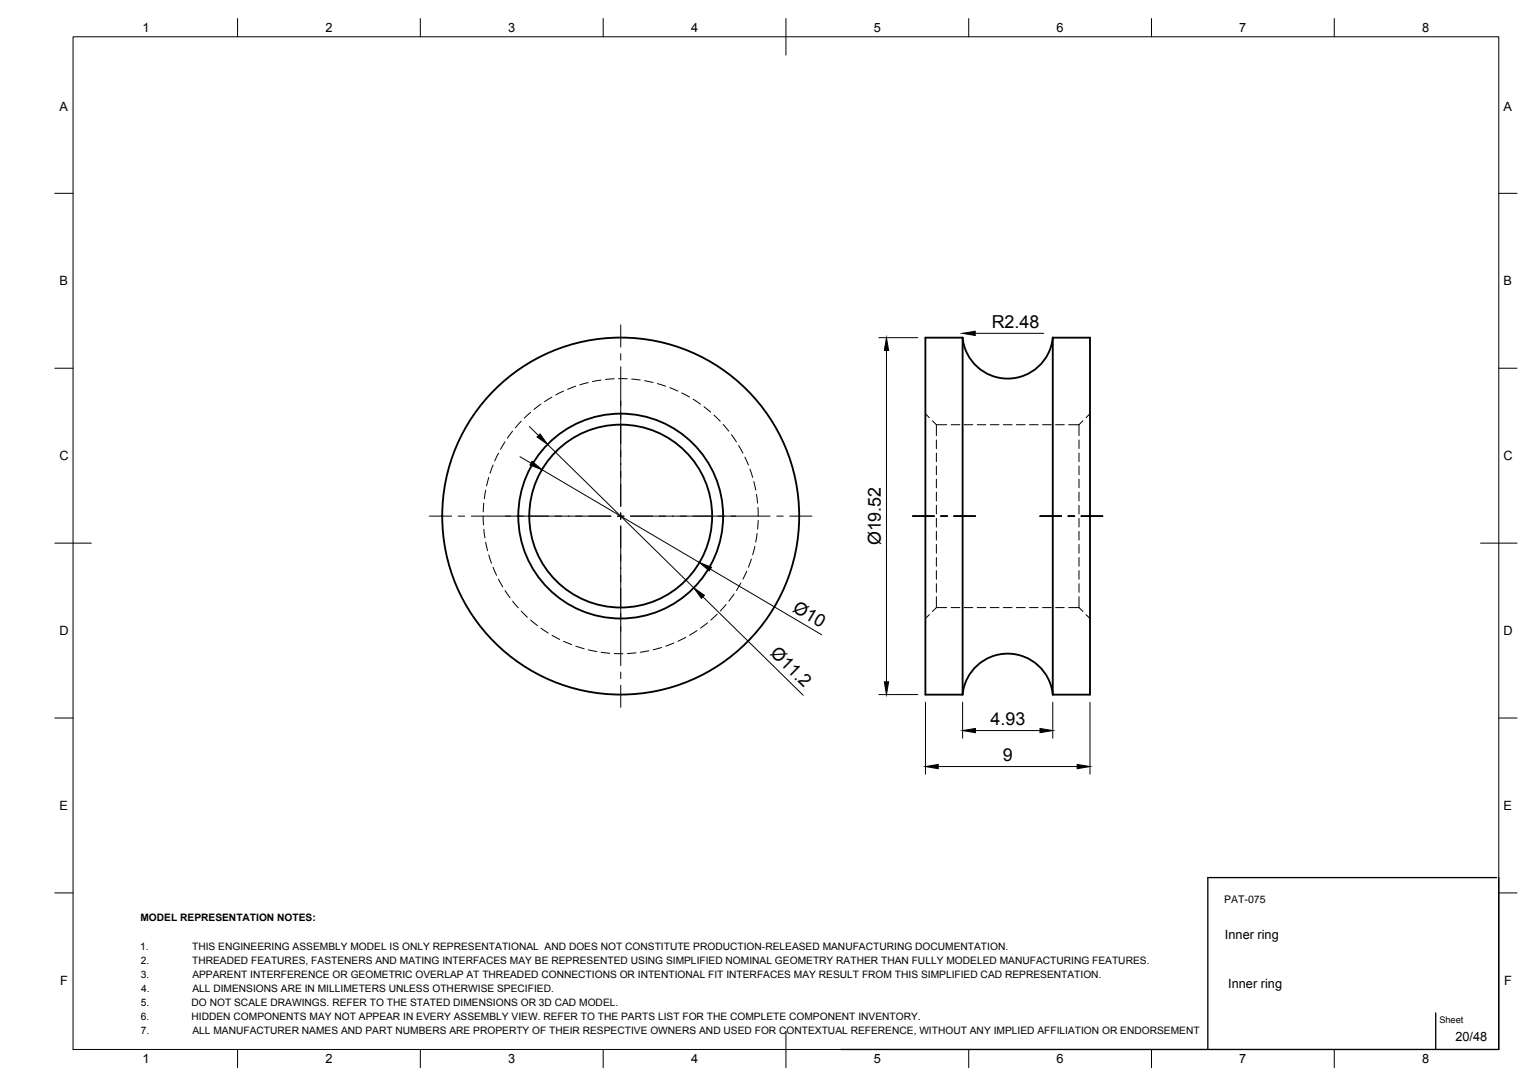
ISO-10303-21;
HEADER;
/* Generated by software containing ST-Developer
 * from STEP Tools, Inc. (www.steptools.com) 
 */

FILE_DESCRIPTION(
/* description */ ('Over-Centre Plunger Toggle Clamp on Slotted Fixture Frame'),
/* implementation_level */ '2;1');

FILE_NAME(
/* name */ 
'Inner ring.step',
/* time_stamp */ '2026-10-28T03:23:24-07:00',
/* author */ (''),
/* organization */ (''),
/* preprocessor_version */ 'ST-DEVELOPER v20.2',
/* originating_system */ 'Autodesk Translation Framework v15.17.0.0',
/* authorisation */ '');

FILE_SCHEMA (('AUTOMOTIVE_DESIGN { 1 0 10303 214 3 1 1 }'));
ENDSEC;

DATA;
#10=MECHANICAL_DESIGN_GEOMETRIC_PRESENTATION_REPRESENTATION('',(#529),#15212);
#395=TOROIDAL_SURFACE('',#9166,1.,0.247676);
#409=CONICAL_SURFACE('',#9177,0.53,0.785398163397448);
#410=CONICAL_SURFACE('',#9184,0.53,0.785398163397448);
#445=SHAPE_REPRESENTATION_RELATIONSHIP('SRR','None',#15420,#487);
#487=ADVANCED_BREP_SHAPE_REPRESENTATION('',(#579),#15182);
#529=STYLED_ITEM('',(#15719),#579);
#579=MANIFOLD_SOLID_BREP('Body1',#8262);
#720=FACE_BOUND('',#1918,.T.);
#721=FACE_BOUND('',#1921,.T.);
#938=PLANE('',#9179);
#939=PLANE('',#9182);
#1318=FACE_OUTER_BOUND('',#1913,.T.);
#1319=FACE_OUTER_BOUND('',#1914,.T.);
#1320=FACE_OUTER_BOUND('',#1915,.T.);
#1321=FACE_OUTER_BOUND('',#1916,.T.);
#1322=FACE_OUTER_BOUND('',#1917,.T.);
#1323=FACE_OUTER_BOUND('',#1919,.T.);
#1324=FACE_OUTER_BOUND('',#1920,.T.);
#1325=FACE_OUTER_BOUND('',#1922,.T.);
#1913=EDGE_LOOP('',(#6629,#6630,#6631,#6632,#6633,#6634));
#1914=EDGE_LOOP('',(#6635,#6636,#6637,#6638,#6639));
#1915=EDGE_LOOP('',(#6640,#6641,#6642,#6643));
#1916=EDGE_LOOP('',(#6644,#6645,#6646,#6647));
#1917=EDGE_LOOP('',(#6648));
#1918=EDGE_LOOP('',(#6649));
#1919=EDGE_LOOP('',(#6650,#6651,#6652,#6653,#6654));
#1920=EDGE_LOOP('',(#6655));
#1921=EDGE_LOOP('',(#6656));
#1922=EDGE_LOOP('',(#6657,#6658,#6659,#6660));
#2609=LINE('',#13511,#3239);
#2610=LINE('',#13517,#3240);
#2611=LINE('',#13521,#3241);
#2612=LINE('',#13527,#3242);
#2613=LINE('',#13532,#3243);
#3239=VECTOR('',#10952,0.976185);
#3240=VECTOR('',#10959,0.5);
#3241=VECTOR('',#10964,0.53);
#3242=VECTOR('',#10973,0.976185);
#3243=VECTOR('',#10980,0.53);
#3641=CIRCLE('',#9167,0.976185);
#3642=CIRCLE('',#9168,0.976185);
#3643=CIRCLE('',#9169,0.247676);
#3644=CIRCLE('',#9170,0.976185);
#3645=CIRCLE('',#9171,0.976185);
#3646=CIRCLE('',#9173,0.976185);
#3647=CIRCLE('',#9175,0.5);
#3648=CIRCLE('',#9176,0.5);
#3649=CIRCLE('',#9178,0.56);
#3650=CIRCLE('',#9181,0.976185);
#3651=CIRCLE('',#9183,0.56);
#4211=VERTEX_POINT('',#13500);
#4212=VERTEX_POINT('',#13501);
#4213=VERTEX_POINT('',#13504);
#4214=VERTEX_POINT('',#13506);
#4215=VERTEX_POINT('',#13510);
#4216=VERTEX_POINT('',#13514);
#4217=VERTEX_POINT('',#13516);
#4218=VERTEX_POINT('',#13520);
#4219=VERTEX_POINT('',#13525);
#4220=VERTEX_POINT('',#13529);
#5075=EDGE_CURVE('',#4211,#4212,#3641,.T.);
#5076=EDGE_CURVE('',#4212,#4211,#3642,.T.);
#5077=EDGE_CURVE('',#4212,#4213,#3643,.T.);
#5078=EDGE_CURVE('',#4214,#4213,#3644,.T.);
#5079=EDGE_CURVE('',#4213,#4214,#3645,.T.);
#5080=EDGE_CURVE('',#4214,#4215,#2609,.T.);
#5081=EDGE_CURVE('',#4215,#4215,#3646,.T.);
#5082=EDGE_CURVE('',#4216,#4216,#3647,.T.);
#5083=EDGE_CURVE('',#4216,#4217,#2610,.T.);
#5084=EDGE_CURVE('',#4217,#4217,#3648,.T.);
#5085=EDGE_CURVE('',#4217,#4218,#2611,.T.);
#5086=EDGE_CURVE('',#4218,#4218,#3649,.T.);
#5087=EDGE_CURVE('',#4219,#4219,#3650,.T.);
#5088=EDGE_CURVE('',#4219,#4211,#2612,.T.);
#5089=EDGE_CURVE('',#4220,#4220,#3651,.T.);
#5090=EDGE_CURVE('',#4220,#4216,#2613,.T.);
#6629=ORIENTED_EDGE('',*,*,#5075,.F.);
#6630=ORIENTED_EDGE('',*,*,#5076,.F.);
#6631=ORIENTED_EDGE('',*,*,#5077,.T.);
#6632=ORIENTED_EDGE('',*,*,#5078,.F.);
#6633=ORIENTED_EDGE('',*,*,#5079,.F.);
#6634=ORIENTED_EDGE('',*,*,#5077,.F.);
#6635=ORIENTED_EDGE('',*,*,#5078,.T.);
#6636=ORIENTED_EDGE('',*,*,#5079,.T.);
#6637=ORIENTED_EDGE('',*,*,#5080,.T.);
#6638=ORIENTED_EDGE('',*,*,#5081,.T.);
#6639=ORIENTED_EDGE('',*,*,#5080,.F.);
#6640=ORIENTED_EDGE('',*,*,#5082,.T.);
#6641=ORIENTED_EDGE('',*,*,#5083,.T.);
#6642=ORIENTED_EDGE('',*,*,#5084,.F.);
#6643=ORIENTED_EDGE('',*,*,#5083,.F.);
#6644=ORIENTED_EDGE('',*,*,#5084,.T.);
#6645=ORIENTED_EDGE('',*,*,#5085,.T.);
#6646=ORIENTED_EDGE('',*,*,#5086,.F.);
#6647=ORIENTED_EDGE('',*,*,#5085,.F.);
#6648=ORIENTED_EDGE('',*,*,#5081,.F.);
#6649=ORIENTED_EDGE('',*,*,#5086,.T.);
#6650=ORIENTED_EDGE('',*,*,#5087,.F.);
#6651=ORIENTED_EDGE('',*,*,#5088,.T.);
#6652=ORIENTED_EDGE('',*,*,#5075,.T.);
#6653=ORIENTED_EDGE('',*,*,#5076,.T.);
#6654=ORIENTED_EDGE('',*,*,#5088,.F.);
#6655=ORIENTED_EDGE('',*,*,#5087,.T.);
#6656=ORIENTED_EDGE('',*,*,#5089,.F.);
#6657=ORIENTED_EDGE('',*,*,#5089,.T.);
#6658=ORIENTED_EDGE('',*,*,#5090,.T.);
#6659=ORIENTED_EDGE('',*,*,#5082,.F.);
#6660=ORIENTED_EDGE('',*,*,#5090,.F.);
#7689=CYLINDRICAL_SURFACE('',#9172,0.976185);
#7690=CYLINDRICAL_SURFACE('',#9174,0.5);
#7691=CYLINDRICAL_SURFACE('',#9180,0.976185);
#7990=ADVANCED_FACE('',(#1318),#395,.F.);
#7991=ADVANCED_FACE('',(#1319),#7689,.T.);
#7992=ADVANCED_FACE('',(#1320),#7690,.F.);
#7993=ADVANCED_FACE('',(#1321),#409,.F.);
#7994=ADVANCED_FACE('',(#1322,#720),#938,.T.);
#7995=ADVANCED_FACE('',(#1323),#7691,.T.);
#7996=ADVANCED_FACE('',(#1324,#721),#939,.T.);
#7997=ADVANCED_FACE('',(#1325),#410,.F.);
#8262=CLOSED_SHELL('',(#7990,#7991,#7992,#7993,#7994,#7995,#7996,#7997));
#9165=AXIS2_PLACEMENT_3D('',#13498,#10936,#10937);
#9166=AXIS2_PLACEMENT_3D('',#13499,#10938,#10939);
#9167=AXIS2_PLACEMENT_3D('',#13502,#10940,#10941);
#9168=AXIS2_PLACEMENT_3D('',#13503,#10942,#10943);
#9169=AXIS2_PLACEMENT_3D('',#13505,#10944,#10945);
#9170=AXIS2_PLACEMENT_3D('',#13507,#10946,#10947);
#9171=AXIS2_PLACEMENT_3D('',#13508,#10948,#10949);
#9172=AXIS2_PLACEMENT_3D('',#13509,#10950,#10951);
#9173=AXIS2_PLACEMENT_3D('',#13512,#10953,#10954);
#9174=AXIS2_PLACEMENT_3D('',#13513,#10955,#10956);
#9175=AXIS2_PLACEMENT_3D('',#13515,#10957,#10958);
#9176=AXIS2_PLACEMENT_3D('',#13518,#10960,#10961);
#9177=AXIS2_PLACEMENT_3D('',#13519,#10962,#10963);
#9178=AXIS2_PLACEMENT_3D('',#13522,#10965,#10966);
#9179=AXIS2_PLACEMENT_3D('',#13523,#10967,#10968);
#9180=AXIS2_PLACEMENT_3D('',#13524,#10969,#10970);
#9181=AXIS2_PLACEMENT_3D('',#13526,#10971,#10972);
#9182=AXIS2_PLACEMENT_3D('',#13528,#10974,#10975);
#9183=AXIS2_PLACEMENT_3D('',#13530,#10976,#10977);
#9184=AXIS2_PLACEMENT_3D('',#13531,#10978,#10979);
#10936=DIRECTION('axis',(0.,0.,1.));
#10937=DIRECTION('refdir',(1.,0.,0.));
#10938=DIRECTION('center_axis',(0.,-1.,0.));
#10939=DIRECTION('ref_axis',(0.,0.,-1.));
#10940=DIRECTION('center_axis',(0.,-1.,0.));
#10941=DIRECTION('ref_axis',(1.,0.,0.));
#10942=DIRECTION('center_axis',(0.,-1.,0.));
#10943=DIRECTION('ref_axis',(1.,0.,0.));
#10944=DIRECTION('center_axis',(1.,0.,1.22464679914735E-16));
#10945=DIRECTION('ref_axis',(-1.22464679914735E-16,0.,1.));
#10946=DIRECTION('center_axis',(0.,1.,0.));
#10947=DIRECTION('ref_axis',(1.,0.,0.));
#10948=DIRECTION('center_axis',(0.,1.,0.));
#10949=DIRECTION('ref_axis',(1.,0.,0.));
#10950=DIRECTION('center_axis',(0.,-1.,0.));
#10951=DIRECTION('ref_axis',(1.,0.,0.));
#10952=DIRECTION('',(0.,1.,0.));
#10953=DIRECTION('center_axis',(0.,-1.,0.));
#10954=DIRECTION('ref_axis',(1.,0.,0.));
#10955=DIRECTION('center_axis',(0.,-1.,0.));
#10956=DIRECTION('ref_axis',(1.,0.,0.));
#10957=DIRECTION('center_axis',(0.,-1.,0.));
#10958=DIRECTION('ref_axis',(1.,0.,0.));
#10959=DIRECTION('',(0.,1.,0.));
#10960=DIRECTION('center_axis',(0.,-1.,0.));
#10961=DIRECTION('ref_axis',(1.,0.,0.));
#10962=DIRECTION('center_axis',(0.,1.,0.));
#10963=DIRECTION('ref_axis',(1.,0.,0.));
#10964=DIRECTION('',(-0.707106781186547,0.707106781186548,-8.65956056235493E-17));
#10965=DIRECTION('center_axis',(0.,-1.,0.));
#10966=DIRECTION('ref_axis',(1.,0.,0.));
#10967=DIRECTION('center_axis',(0.,1.,0.));
#10968=DIRECTION('ref_axis',(0.,0.,1.));
#10969=DIRECTION('center_axis',(0.,-1.,0.));
#10970=DIRECTION('ref_axis',(1.,0.,0.));
#10971=DIRECTION('center_axis',(0.,-1.,0.));
#10972=DIRECTION('ref_axis',(1.,0.,0.));
#10973=DIRECTION('',(0.,1.,0.));
#10974=DIRECTION('center_axis',(0.,-1.,0.));
#10975=DIRECTION('ref_axis',(0.,0.,-1.));
#10976=DIRECTION('center_axis',(0.,-1.,0.));
#10977=DIRECTION('ref_axis',(1.,0.,0.));
#10978=DIRECTION('center_axis',(0.,-1.,0.));
#10979=DIRECTION('ref_axis',(1.,0.,0.));
#10980=DIRECTION('',(0.707106781186547,0.707106781186548,8.65956056235493E-17));
#13498=CARTESIAN_POINT('',(0.,0.,0.));
#13499=CARTESIAN_POINT('Origin',(0.,0.,0.));
#13500=CARTESIAN_POINT('',(-0.976185,-0.246528389340863,-1.19548183562566E-16));
#13501=CARTESIAN_POINT('',(-1.19548183562566E-16,-0.246528389340863,0.976185));
#13502=CARTESIAN_POINT('Origin',(0.,-0.246528389340863,0.));
#13503=CARTESIAN_POINT('Origin',(0.,-0.246528389340863,0.));
#13504=CARTESIAN_POINT('',(-1.19548183562566E-16,0.246528389340863,0.976185));
#13505=CARTESIAN_POINT('Origin',(-1.22464679914735E-16,0.,1.));
#13506=CARTESIAN_POINT('',(-0.976185,0.246528389340863,1.19548183562566E-16));
#13507=CARTESIAN_POINT('Origin',(0.,0.246528389340863,0.));
#13508=CARTESIAN_POINT('Origin',(0.,0.246528389340863,0.));
#13509=CARTESIAN_POINT('Origin',(0.,0.,0.));
#13510=CARTESIAN_POINT('',(-0.976185,0.45,-1.19548183562566E-16));
#13511=CARTESIAN_POINT('',(-0.976185,0.,-1.19548183562566E-16));
#13512=CARTESIAN_POINT('Origin',(0.,0.45,0.));
#13513=CARTESIAN_POINT('Origin',(0.,0.,0.));
#13514=CARTESIAN_POINT('',(-0.5,-0.39,-6.12323399573677E-17));
#13515=CARTESIAN_POINT('Origin',(0.,-0.39,0.));
#13516=CARTESIAN_POINT('',(-0.5,0.39,-6.12323399573677E-17));
#13517=CARTESIAN_POINT('',(-0.5,0.,-6.12323399573677E-17));
#13518=CARTESIAN_POINT('Origin',(0.,0.39,0.));
#13519=CARTESIAN_POINT('Origin',(0.,0.42,0.));
#13520=CARTESIAN_POINT('',(-0.56,0.45,-6.85802207522518E-17));
#13521=CARTESIAN_POINT('',(-0.53,0.42,-6.49062803548097E-17));
#13522=CARTESIAN_POINT('Origin',(0.,0.45,0.));
#13523=CARTESIAN_POINT('Origin',(0.976185,0.45,0.));
#13524=CARTESIAN_POINT('Origin',(0.,0.,0.));
#13525=CARTESIAN_POINT('',(-0.976185,-0.45,-1.19548183562566E-16));
#13526=CARTESIAN_POINT('Origin',(0.,-0.45,0.));
#13527=CARTESIAN_POINT('',(-0.976185,0.,-1.19548183562566E-16));
#13528=CARTESIAN_POINT('Origin',(0.56,-0.45,0.));
#13529=CARTESIAN_POINT('',(-0.56,-0.45,-6.85802207522518E-17));
#13530=CARTESIAN_POINT('Origin',(0.,-0.45,0.));
#13531=CARTESIAN_POINT('Origin',(0.,-0.42,0.));
#13532=CARTESIAN_POINT('',(-0.53,-0.42,-6.49062803548097E-17));
#15132=UNCERTAINTY_MEASURE_WITH_UNIT(LENGTH_MEASURE(0.001),#15213,
'DISTANCE_ACCURACY_VALUE',
'Maximum model space distance between geometric entities at asserted c
onnectivities');
#15162=UNCERTAINTY_MEASURE_WITH_UNIT(LENGTH_MEASURE(0.001),#15213,
'DISTANCE_ACCURACY_VALUE',
'Maximum model space distance between geometric entities at asserted c
onnectivities');
#15182=(
GEOMETRIC_REPRESENTATION_CONTEXT(3)
GLOBAL_UNCERTAINTY_ASSIGNED_CONTEXT((#15132))
GLOBAL_UNIT_ASSIGNED_CONTEXT((#15213,#15215,#15216))
REPRESENTATION_CONTEXT('','3D')
);
#15212=(
GEOMETRIC_REPRESENTATION_CONTEXT(3)
GLOBAL_UNCERTAINTY_ASSIGNED_CONTEXT((#15162))
GLOBAL_UNIT_ASSIGNED_CONTEXT((#15213,#15215,#15216))
REPRESENTATION_CONTEXT('','3D')
);
#15213=(
LENGTH_UNIT()
NAMED_UNIT(*)
SI_UNIT(.CENTI.,.METRE.)
);
#15215=(
NAMED_UNIT(*)
PLANE_ANGLE_UNIT()
SI_UNIT($,.RADIAN.)
);
#15216=(
NAMED_UNIT(*)
SI_UNIT($,.STERADIAN.)
SOLID_ANGLE_UNIT()
);
#15236=SHAPE_DEFINITION_REPRESENTATION(#15285,#15420);
#15285=PRODUCT_DEFINITION_SHAPE('',$,#15470);
#15420=SHAPE_REPRESENTATION('',(#9165),#15182);
#15450=PRODUCT_DEFINITION_CONTEXT('part definition',#15599,'design');
#15470=PRODUCT_DEFINITION('Inner ring','Inner ring',#15519,#15450);
#15519=PRODUCT_DEFINITION_FORMATION('',$,#15620);
#15599=APPLICATION_CONTEXT(
'Core Data for Automotive Mechanical Design Process');
#15600=PRODUCT_CONTEXT('part definition',#15599,'mechanical');
#15620=PRODUCT('Inner ring','Inner ring','Inner ring',(#15600));
#15713=COLOUR_RGB('Grey',0.48,0.52,0.57);
#15714=FILL_AREA_STYLE_COLOUR('',#15713);
#15715=FILL_AREA_STYLE('',(#15714));
#15716=SURFACE_STYLE_FILL_AREA(#15715);
#15717=SURFACE_SIDE_STYLE('',(#15716));
#15718=SURFACE_STYLE_USAGE(.BOTH.,#15717);
#15719=PRESENTATION_STYLE_ASSIGNMENT((#15718));
ENDSEC;
END-ISO-10303-21;
